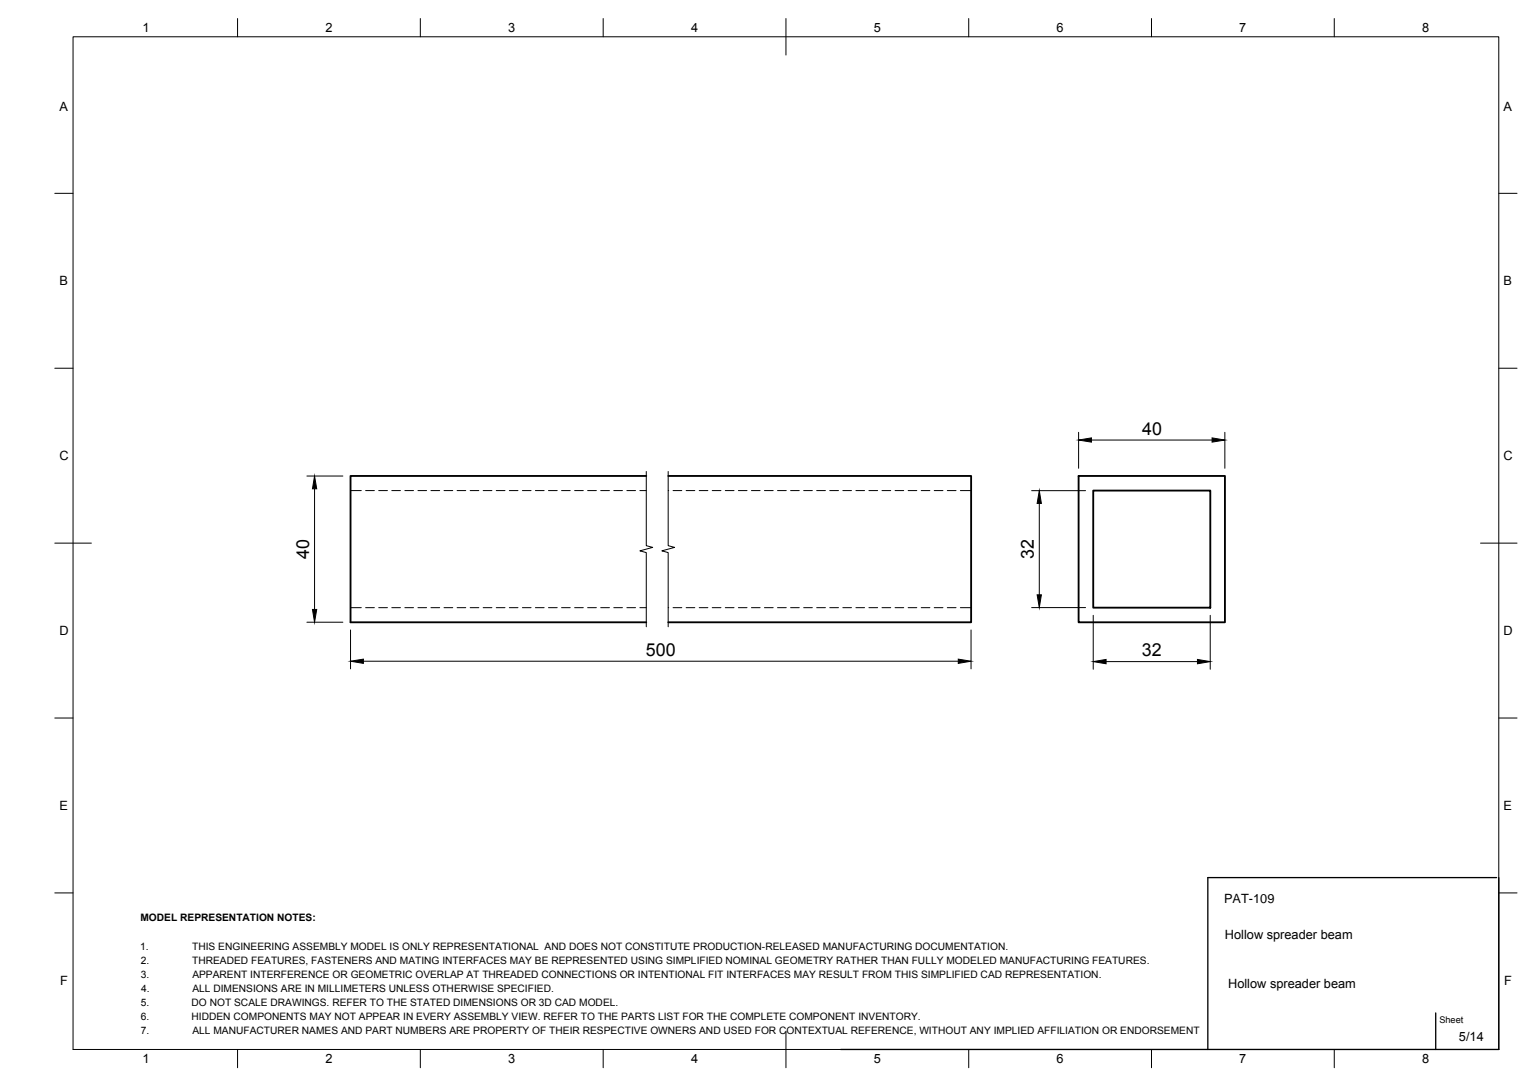
ISO-10303-21;
HEADER;
/* Generated by software containing ST-Developer
 * from STEP Tools, Inc. (www.steptools.com) 
 */

FILE_DESCRIPTION(
/* description */ ('Twin-shackle spreader bar'),
/* implementation_level */ '2;1');

FILE_NAME(
/* name */ 'Hollow spreader beam.step',
/* time_stamp */ '2026-10-27T20:18:10-07:00',
/* author */ (''),
/* organization */ (''),
/* preprocessor_version */ 'ST-DEVELOPER v20.2',
/* originating_system */ 'Autodesk Translation Framework v15.17.0.0',
/* authorisation */ '');

FILE_SCHEMA (('AUTOMOTIVE_DESIGN { 1 0 10303 214 3 1 1 }'));
ENDSEC;

DATA;
#10=MECHANICAL_DESIGN_GEOMETRIC_PRESENTATION_REPRESENTATION('',(#157),#1829);
#143=SHAPE_REPRESENTATION_RELATIONSHIP('SRR','None',#1879,#150);
#150=ADVANCED_BREP_SHAPE_REPRESENTATION('',(#164),#1820);
#157=STYLED_ITEM('',(#1977),#164);
#164=MANIFOLD_SOLID_BREP('Body1',#937);
#171=FACE_BOUND('',#242,.T.);
#172=FACE_BOUND('',#245,.T.);
#186=FACE_OUTER_BOUND('',#236,.T.);
#187=FACE_OUTER_BOUND('',#237,.T.);
#188=FACE_OUTER_BOUND('',#238,.T.);
#189=FACE_OUTER_BOUND('',#239,.T.);
#190=FACE_OUTER_BOUND('',#240,.T.);
#191=FACE_OUTER_BOUND('',#241,.T.);
#192=FACE_OUTER_BOUND('',#243,.T.);
#193=FACE_OUTER_BOUND('',#244,.T.);
#194=FACE_OUTER_BOUND('',#246,.T.);
#195=FACE_OUTER_BOUND('',#247,.T.);
#236=EDGE_LOOP('',(#634,#635,#636,#637));
#237=EDGE_LOOP('',(#638,#639,#640,#641));
#238=EDGE_LOOP('',(#642,#643,#644,#645));
#239=EDGE_LOOP('',(#646,#647,#648,#649));
#240=EDGE_LOOP('',(#650,#651,#652,#653));
#241=EDGE_LOOP('',(#654,#655,#656,#657));
#242=EDGE_LOOP('',(#658,#659,#660,#661));
#243=EDGE_LOOP('',(#662,#663,#664,#665));
#244=EDGE_LOOP('',(#666,#667,#668,#669));
#245=EDGE_LOOP('',(#670,#671,#672,#673));
#246=EDGE_LOOP('',(#674,#675,#676,#677));
#247=EDGE_LOOP('',(#678,#679,#680,#681));
#301=LINE('',#1431,#377);
#302=LINE('',#1433,#378);
#303=LINE('',#1435,#379);
#304=LINE('',#1436,#380);
#305=LINE('',#1439,#381);
#306=LINE('',#1441,#382);
#307=LINE('',#1442,#383);
#308=LINE('',#1445,#384);
#309=LINE('',#1447,#385);
#310=LINE('',#1448,#386);
#311=LINE('',#1450,#387);
#312=LINE('',#1451,#388);
#313=LINE('',#1455,#389);
#314=LINE('',#1457,#390);
#315=LINE('',#1459,#391);
#316=LINE('',#1460,#392);
#317=LINE('',#1463,#393);
#318=LINE('',#1465,#394);
#319=LINE('',#1466,#395);
#320=LINE('',#1469,#396);
#321=LINE('',#1471,#397);
#322=LINE('',#1472,#398);
#323=LINE('',#1474,#399);
#324=LINE('',#1475,#400);
#377=VECTOR('',#1139,1.);
#378=VECTOR('',#1140,1.);
#379=VECTOR('',#1141,1.);
#380=VECTOR('',#1142,1.);
#381=VECTOR('',#1145,1.);
#382=VECTOR('',#1146,1.);
#383=VECTOR('',#1147,1.);
#384=VECTOR('',#1150,1.);
#385=VECTOR('',#1151,1.);
#386=VECTOR('',#1152,1.);
#387=VECTOR('',#1155,1.);
#388=VECTOR('',#1156,1.);
#389=VECTOR('',#1159,1.);
#390=VECTOR('',#1160,1.);
#391=VECTOR('',#1161,1.);
#392=VECTOR('',#1162,1.);
#393=VECTOR('',#1165,1.);
#394=VECTOR('',#1166,1.);
#395=VECTOR('',#1167,1.);
#396=VECTOR('',#1170,1.);
#397=VECTOR('',#1171,1.);
#398=VECTOR('',#1172,1.);
#399=VECTOR('',#1175,1.);
#400=VECTOR('',#1176,1.);
#453=VERTEX_POINT('',#1429);
#454=VERTEX_POINT('',#1430);
#455=VERTEX_POINT('',#1432);
#456=VERTEX_POINT('',#1434);
#457=VERTEX_POINT('',#1438);
#458=VERTEX_POINT('',#1440);
#459=VERTEX_POINT('',#1444);
#460=VERTEX_POINT('',#1446);
#461=VERTEX_POINT('',#1453);
#462=VERTEX_POINT('',#1454);
#463=VERTEX_POINT('',#1456);
#464=VERTEX_POINT('',#1458);
#465=VERTEX_POINT('',#1462);
#466=VERTEX_POINT('',#1464);
#467=VERTEX_POINT('',#1468);
#468=VERTEX_POINT('',#1470);
#525=EDGE_CURVE('',#453,#454,#301,.T.);
#526=EDGE_CURVE('',#455,#453,#302,.T.);
#527=EDGE_CURVE('',#456,#455,#303,.T.);
#528=EDGE_CURVE('',#456,#454,#304,.T.);
#529=EDGE_CURVE('',#454,#457,#305,.T.);
#530=EDGE_CURVE('',#458,#456,#306,.T.);
#531=EDGE_CURVE('',#458,#457,#307,.T.);
#532=EDGE_CURVE('',#457,#459,#308,.T.);
#533=EDGE_CURVE('',#460,#458,#309,.T.);
#534=EDGE_CURVE('',#460,#459,#310,.T.);
#535=EDGE_CURVE('',#459,#453,#311,.T.);
#536=EDGE_CURVE('',#455,#460,#312,.T.);
#537=EDGE_CURVE('',#461,#462,#313,.T.);
#538=EDGE_CURVE('',#462,#463,#314,.T.);
#539=EDGE_CURVE('',#464,#463,#315,.T.);
#540=EDGE_CURVE('',#461,#464,#316,.T.);
#541=EDGE_CURVE('',#465,#461,#317,.T.);
#542=EDGE_CURVE('',#466,#464,#318,.T.);
#543=EDGE_CURVE('',#465,#466,#319,.T.);
#544=EDGE_CURVE('',#467,#465,#320,.T.);
#545=EDGE_CURVE('',#468,#466,#321,.T.);
#546=EDGE_CURVE('',#467,#468,#322,.T.);
#547=EDGE_CURVE('',#462,#467,#323,.T.);
#548=EDGE_CURVE('',#463,#468,#324,.T.);
#634=ORIENTED_EDGE('',*,*,#525,.F.);
#635=ORIENTED_EDGE('',*,*,#526,.F.);
#636=ORIENTED_EDGE('',*,*,#527,.F.);
#637=ORIENTED_EDGE('',*,*,#528,.T.);
#638=ORIENTED_EDGE('',*,*,#529,.F.);
#639=ORIENTED_EDGE('',*,*,#528,.F.);
#640=ORIENTED_EDGE('',*,*,#530,.F.);
#641=ORIENTED_EDGE('',*,*,#531,.T.);
#642=ORIENTED_EDGE('',*,*,#532,.F.);
#643=ORIENTED_EDGE('',*,*,#531,.F.);
#644=ORIENTED_EDGE('',*,*,#533,.F.);
#645=ORIENTED_EDGE('',*,*,#534,.T.);
#646=ORIENTED_EDGE('',*,*,#535,.F.);
#647=ORIENTED_EDGE('',*,*,#534,.F.);
#648=ORIENTED_EDGE('',*,*,#536,.F.);
#649=ORIENTED_EDGE('',*,*,#526,.T.);
#650=ORIENTED_EDGE('',*,*,#537,.T.);
#651=ORIENTED_EDGE('',*,*,#538,.T.);
#652=ORIENTED_EDGE('',*,*,#539,.F.);
#653=ORIENTED_EDGE('',*,*,#540,.F.);
#654=ORIENTED_EDGE('',*,*,#541,.T.);
#655=ORIENTED_EDGE('',*,*,#540,.T.);
#656=ORIENTED_EDGE('',*,*,#542,.F.);
#657=ORIENTED_EDGE('',*,*,#543,.F.);
#658=ORIENTED_EDGE('',*,*,#532,.T.);
#659=ORIENTED_EDGE('',*,*,#535,.T.);
#660=ORIENTED_EDGE('',*,*,#525,.T.);
#661=ORIENTED_EDGE('',*,*,#529,.T.);
#662=ORIENTED_EDGE('',*,*,#544,.T.);
#663=ORIENTED_EDGE('',*,*,#543,.T.);
#664=ORIENTED_EDGE('',*,*,#545,.F.);
#665=ORIENTED_EDGE('',*,*,#546,.F.);
#666=ORIENTED_EDGE('',*,*,#547,.T.);
#667=ORIENTED_EDGE('',*,*,#546,.T.);
#668=ORIENTED_EDGE('',*,*,#548,.F.);
#669=ORIENTED_EDGE('',*,*,#538,.F.);
#670=ORIENTED_EDGE('',*,*,#533,.T.);
#671=ORIENTED_EDGE('',*,*,#530,.T.);
#672=ORIENTED_EDGE('',*,*,#527,.T.);
#673=ORIENTED_EDGE('',*,*,#536,.T.);
#674=ORIENTED_EDGE('',*,*,#548,.T.);
#675=ORIENTED_EDGE('',*,*,#545,.T.);
#676=ORIENTED_EDGE('',*,*,#542,.T.);
#677=ORIENTED_EDGE('',*,*,#539,.T.);
#678=ORIENTED_EDGE('',*,*,#547,.F.);
#679=ORIENTED_EDGE('',*,*,#537,.F.);
#680=ORIENTED_EDGE('',*,*,#541,.F.);
#681=ORIENTED_EDGE('',*,*,#544,.F.);
#852=PLANE('',#1025);
#853=PLANE('',#1026);
#854=PLANE('',#1027);
#855=PLANE('',#1028);
#856=PLANE('',#1029);
#857=PLANE('',#1030);
#858=PLANE('',#1031);
#859=PLANE('',#1032);
#860=PLANE('',#1033);
#861=PLANE('',#1034);
#887=ADVANCED_FACE('',(#186),#852,.F.);
#888=ADVANCED_FACE('',(#187),#853,.F.);
#889=ADVANCED_FACE('',(#188),#854,.F.);
#890=ADVANCED_FACE('',(#189),#855,.F.);
#891=ADVANCED_FACE('',(#190),#856,.T.);
#892=ADVANCED_FACE('',(#191,#171),#857,.T.);
#893=ADVANCED_FACE('',(#192),#858,.T.);
#894=ADVANCED_FACE('',(#193,#172),#859,.T.);
#895=ADVANCED_FACE('',(#194),#860,.T.);
#896=ADVANCED_FACE('',(#195),#861,.F.);
#937=CLOSED_SHELL('',(#887,#888,#889,#890,#891,#892,#893,#894,#895,#896));
#1024=AXIS2_PLACEMENT_3D('',#1427,#1135,#1136);
#1025=AXIS2_PLACEMENT_3D('',#1428,#1137,#1138);
#1026=AXIS2_PLACEMENT_3D('',#1437,#1143,#1144);
#1027=AXIS2_PLACEMENT_3D('',#1443,#1148,#1149);
#1028=AXIS2_PLACEMENT_3D('',#1449,#1153,#1154);
#1029=AXIS2_PLACEMENT_3D('',#1452,#1157,#1158);
#1030=AXIS2_PLACEMENT_3D('',#1461,#1163,#1164);
#1031=AXIS2_PLACEMENT_3D('',#1467,#1168,#1169);
#1032=AXIS2_PLACEMENT_3D('',#1473,#1173,#1174);
#1033=AXIS2_PLACEMENT_3D('',#1476,#1177,#1178);
#1034=AXIS2_PLACEMENT_3D('',#1477,#1179,#1180);
#1135=DIRECTION('axis',(0.,0.,1.));
#1136=DIRECTION('refdir',(1.,0.,0.));
#1137=DIRECTION('center_axis',(0.,0.,-1.));
#1138=DIRECTION('ref_axis',(0.,1.,0.));
#1139=DIRECTION('',(0.,-1.,0.));
#1140=DIRECTION('',(1.,0.,0.));
#1141=DIRECTION('',(0.,1.,0.));
#1142=DIRECTION('',(1.,0.,0.));
#1143=DIRECTION('center_axis',(0.,-1.,0.));
#1144=DIRECTION('ref_axis',(0.,0.,-1.));
#1145=DIRECTION('',(0.,0.,1.));
#1146=DIRECTION('',(0.,0.,-1.));
#1147=DIRECTION('',(1.,0.,0.));
#1148=DIRECTION('center_axis',(0.,0.,1.));
#1149=DIRECTION('ref_axis',(0.,-1.,0.));
#1150=DIRECTION('',(0.,1.,0.));
#1151=DIRECTION('',(0.,-1.,0.));
#1152=DIRECTION('',(1.,0.,0.));
#1153=DIRECTION('center_axis',(0.,1.,0.));
#1154=DIRECTION('ref_axis',(0.,0.,1.));
#1155=DIRECTION('',(0.,0.,-1.));
#1156=DIRECTION('',(0.,0.,1.));
#1157=DIRECTION('center_axis',(0.,1.,0.));
#1158=DIRECTION('ref_axis',(-1.,0.,0.));
#1159=DIRECTION('',(-1.,0.,0.));
#1160=DIRECTION('',(0.,0.,1.));
#1161=DIRECTION('',(-1.,0.,0.));
#1162=DIRECTION('',(0.,0.,1.));
#1163=DIRECTION('center_axis',(1.,0.,0.));
#1164=DIRECTION('ref_axis',(0.,1.,0.));
#1165=DIRECTION('',(0.,1.,0.));
#1166=DIRECTION('',(0.,1.,0.));
#1167=DIRECTION('',(0.,0.,1.));
#1168=DIRECTION('center_axis',(0.,-1.,0.));
#1169=DIRECTION('ref_axis',(1.,0.,0.));
#1170=DIRECTION('',(1.,0.,0.));
#1171=DIRECTION('',(1.,0.,0.));
#1172=DIRECTION('',(0.,0.,1.));
#1173=DIRECTION('center_axis',(-1.,0.,0.));
#1174=DIRECTION('ref_axis',(0.,-1.,0.));
#1175=DIRECTION('',(0.,-1.,0.));
#1176=DIRECTION('',(0.,-1.,0.));
#1177=DIRECTION('center_axis',(0.,0.,1.));
#1178=DIRECTION('ref_axis',(1.,0.,0.));
#1179=DIRECTION('center_axis',(0.,0.,1.));
#1180=DIRECTION('ref_axis',(1.,0.,0.));
#1427=CARTESIAN_POINT('',(0.,0.,0.));
#1428=CARTESIAN_POINT('Origin',(-25.1,-1.6,0.4));
#1429=CARTESIAN_POINT('',(25.,1.6,0.4));
#1430=CARTESIAN_POINT('',(25.,-1.6,0.4));
#1431=CARTESIAN_POINT('',(25.,-1.8,0.4));
#1432=CARTESIAN_POINT('',(-25.,1.6,0.4));
#1433=CARTESIAN_POINT('',(-25.1,1.6,0.4));
#1434=CARTESIAN_POINT('',(-25.,-1.6,0.4));
#1435=CARTESIAN_POINT('',(-25.,0.2,0.4));
#1436=CARTESIAN_POINT('',(-25.1,-1.6,0.4));
#1437=CARTESIAN_POINT('Origin',(-25.1,-1.6,3.6));
#1438=CARTESIAN_POINT('',(25.,-1.6,3.6));
#1439=CARTESIAN_POINT('',(25.,-1.6,1.8));
#1440=CARTESIAN_POINT('',(-25.,-1.6,3.6));
#1441=CARTESIAN_POINT('',(-25.,-1.6,1.8));
#1442=CARTESIAN_POINT('',(-25.1,-1.6,3.6));
#1443=CARTESIAN_POINT('Origin',(-25.1,1.6,3.6));
#1444=CARTESIAN_POINT('',(25.,1.6,3.6));
#1445=CARTESIAN_POINT('',(25.,-0.2,3.6));
#1446=CARTESIAN_POINT('',(-25.,1.6,3.6));
#1447=CARTESIAN_POINT('',(-25.,1.8,3.6));
#1448=CARTESIAN_POINT('',(-25.1,1.6,3.6));
#1449=CARTESIAN_POINT('Origin',(-25.1,1.6,0.4));
#1450=CARTESIAN_POINT('',(25.,1.6,0.2));
#1451=CARTESIAN_POINT('',(-25.,1.6,0.2));
#1452=CARTESIAN_POINT('Origin',(25.,2.,0.));
#1453=CARTESIAN_POINT('',(25.,2.,0.));
#1454=CARTESIAN_POINT('',(-25.,2.,0.));
#1455=CARTESIAN_POINT('',(25.,2.,0.));
#1456=CARTESIAN_POINT('',(-25.,2.,4.));
#1457=CARTESIAN_POINT('',(-25.,2.,0.));
#1458=CARTESIAN_POINT('',(25.,2.,4.));
#1459=CARTESIAN_POINT('',(25.,2.,4.));
#1460=CARTESIAN_POINT('',(25.,2.,0.));
#1461=CARTESIAN_POINT('Origin',(25.,-2.,0.));
#1462=CARTESIAN_POINT('',(25.,-2.,0.));
#1463=CARTESIAN_POINT('',(25.,-2.,0.));
#1464=CARTESIAN_POINT('',(25.,-2.,4.));
#1465=CARTESIAN_POINT('',(25.,-2.,4.));
#1466=CARTESIAN_POINT('',(25.,-2.,0.));
#1467=CARTESIAN_POINT('Origin',(-25.,-2.,0.));
#1468=CARTESIAN_POINT('',(-25.,-2.,0.));
#1469=CARTESIAN_POINT('',(-25.,-2.,0.));
#1470=CARTESIAN_POINT('',(-25.,-2.,4.));
#1471=CARTESIAN_POINT('',(-25.,-2.,4.));
#1472=CARTESIAN_POINT('',(-25.,-2.,0.));
#1473=CARTESIAN_POINT('Origin',(-25.,2.,0.));
#1474=CARTESIAN_POINT('',(-25.,2.,0.));
#1475=CARTESIAN_POINT('',(-25.,2.,4.));
#1476=CARTESIAN_POINT('Origin',(0.,0.,4.));
#1477=CARTESIAN_POINT('Origin',(0.,0.,0.));
#1808=UNCERTAINTY_MEASURE_WITH_UNIT(LENGTH_MEASURE(0.001),#1830,
'DISTANCE_ACCURACY_VALUE',
'Maximum model space distance between geometric entities at asserted c
onnectivities');
#1817=UNCERTAINTY_MEASURE_WITH_UNIT(LENGTH_MEASURE(0.001),#1830,
'DISTANCE_ACCURACY_VALUE',
'Maximum model space distance between geometric entities at asserted c
onnectivities');
#1820=(
GEOMETRIC_REPRESENTATION_CONTEXT(3)
GLOBAL_UNCERTAINTY_ASSIGNED_CONTEXT((#1808))
GLOBAL_UNIT_ASSIGNED_CONTEXT((#1830,#1832,#1833))
REPRESENTATION_CONTEXT('','3D')
);
#1829=(
GEOMETRIC_REPRESENTATION_CONTEXT(3)
GLOBAL_UNCERTAINTY_ASSIGNED_CONTEXT((#1817))
GLOBAL_UNIT_ASSIGNED_CONTEXT((#1830,#1832,#1833))
REPRESENTATION_CONTEXT('','3D')
);
#1830=(
LENGTH_UNIT()
NAMED_UNIT(*)
SI_UNIT(.CENTI.,.METRE.)
);
#1832=(
NAMED_UNIT(*)
PLANE_ANGLE_UNIT()
SI_UNIT($,.RADIAN.)
);
#1833=(
NAMED_UNIT(*)
SI_UNIT($,.STERADIAN.)
SOLID_ANGLE_UNIT()
);
#1836=SHAPE_DEFINITION_REPRESENTATION(#1847,#1879);
#1847=PRODUCT_DEFINITION_SHAPE('',$,#1891);
#1879=SHAPE_REPRESENTATION('',(#1024),#1820);
#1888=PRODUCT_DEFINITION_CONTEXT('part definition',#1923,'design');
#1891=PRODUCT_DEFINITION('Hollow spreader beam','Hollow spreader beam',
#1902,#1888);
#1902=PRODUCT_DEFINITION_FORMATION('',$,#1927);
#1923=APPLICATION_CONTEXT(
'Core Data for Automotive Mechanical Design Process');
#1924=PRODUCT_CONTEXT('part definition',#1923,'mechanical');
#1927=PRODUCT('Hollow spreader beam','Hollow spreader beam',
'Hollow spreader beam',(#1924));
#1971=COLOUR_RGB('Sky Blue',0.24,0.69,0.87);
#1972=FILL_AREA_STYLE_COLOUR('',#1971);
#1973=FILL_AREA_STYLE('',(#1972));
#1974=SURFACE_STYLE_FILL_AREA(#1973);
#1975=SURFACE_SIDE_STYLE('',(#1974));
#1976=SURFACE_STYLE_USAGE(.BOTH.,#1975);
#1977=PRESENTATION_STYLE_ASSIGNMENT((#1976));
ENDSEC;
END-ISO-10303-21;
